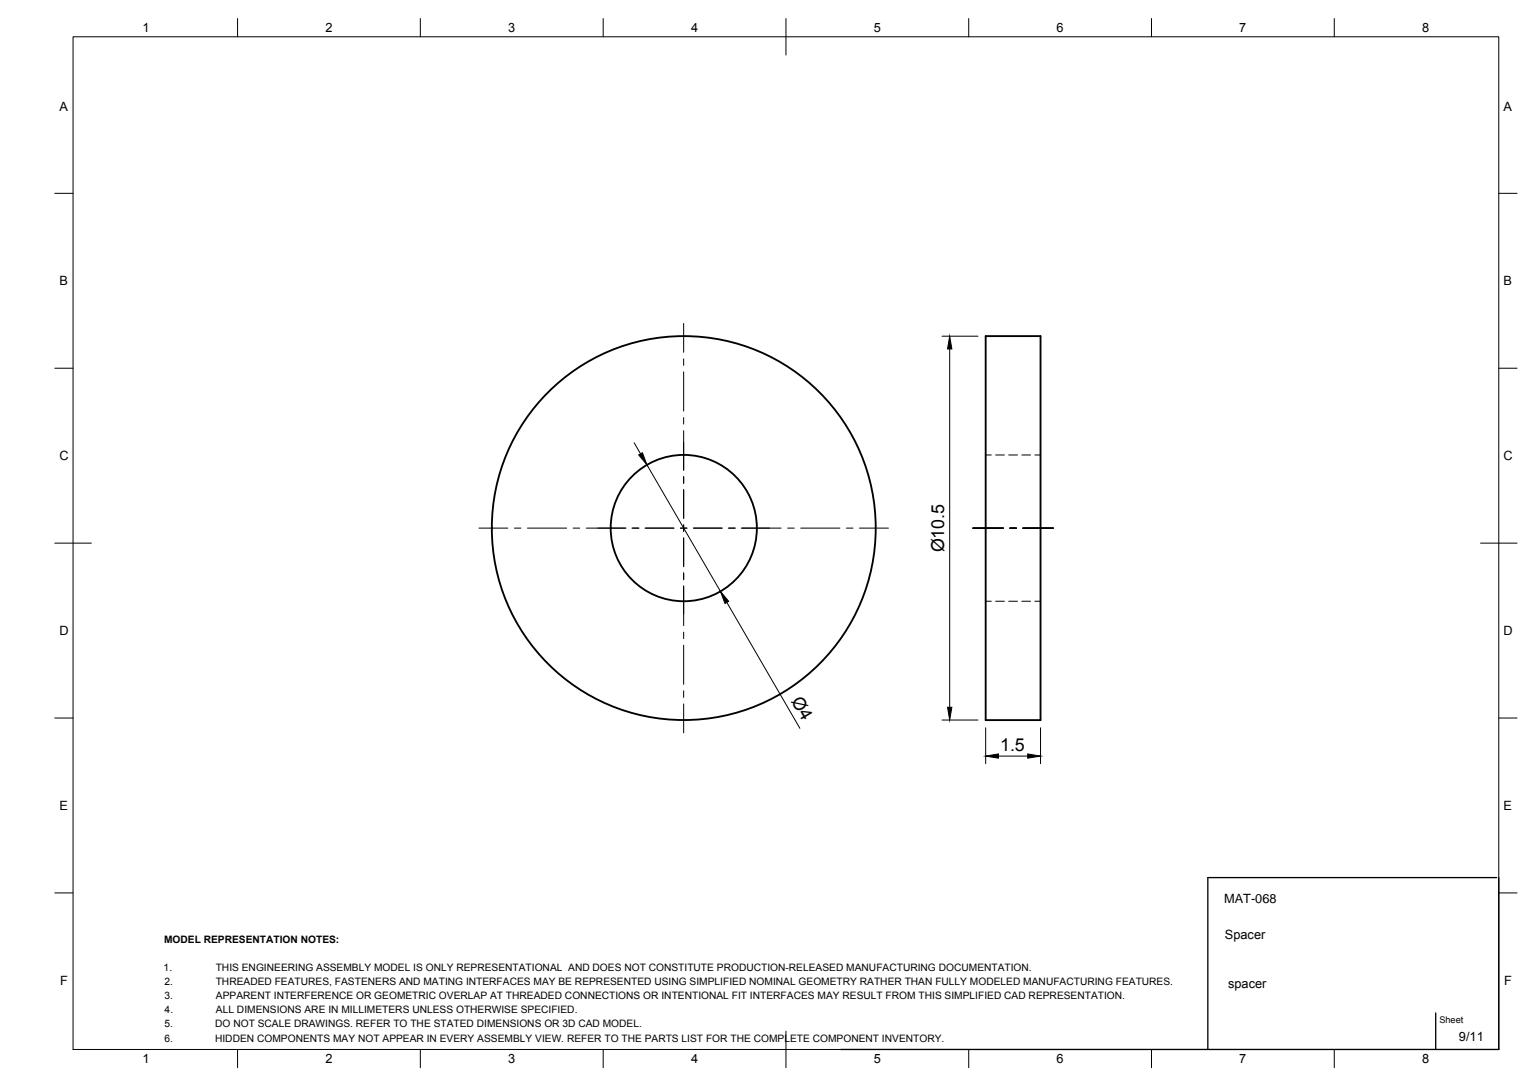
ISO-10303-21;
HEADER;
/* Generated by software containing ST-Developer
 * from STEP Tools, Inc. (www.steptools.com) 
 */

FILE_DESCRIPTION(
/* description */ ('CAx-IF Rec.Pracs.---Representation and Presentation of Product Manufa
cturing Information (PMI)---4.0---2014-10-13'),
/* implementation_level */ '2;1');

FILE_NAME(
/* name */ 'Spacer.step',
/* time_stamp */ '2026-10-24T16:53:48-07:00',
/* author */ (''),
/* organization */ (''),
/* preprocessor_version */ 'ST-DEVELOPER v20.2',
/* originating_system */ 'Autodesk Translation Framework v15.17.0.0',
/* authorisation */ '');

FILE_SCHEMA (('AP242_MANAGED_MODEL_BASED_3D_ENGINEERING_MIM_LF { 1 0 10303 442 2 1 4 }'));
ENDSEC;

DATA;
#10=MECHANICAL_DESIGN_GEOMETRIC_PRESENTATION_REPRESENTATION('',(#3496),#107910);
#3476=SHAPE_REPRESENTATION_RELATIONSHIP('SRR','None',#107954,#3486);
#3486=ADVANCED_BREP_SHAPE_REPRESENTATION('',(#3506),#107907);
#3496=STYLED_ITEM('',(#108011),#3506);
#3506=MANIFOLD_SOLID_BREP('Body1',#45544);
#3517=FACE_BOUND('',#9340,.T.);
#3518=FACE_BOUND('',#9342,.T.);
#3572=PLANE('',#49897);
#3573=PLANE('',#49898);
#6405=FACE_OUTER_BOUND('',#9337,.T.);
#6406=FACE_OUTER_BOUND('',#9338,.T.);
#6407=FACE_OUTER_BOUND('',#9339,.T.);
#6408=FACE_OUTER_BOUND('',#9341,.T.);
#9337=EDGE_LOOP('',(#40400,#40401,#40402,#40403));
#9338=EDGE_LOOP('',(#40404,#40405,#40406,#40407));
#9339=EDGE_LOOP('',(#40408));
#9340=EDGE_LOOP('',(#40409));
#9341=EDGE_LOOP('',(#40410));
#9342=EDGE_LOOP('',(#40411));
#11042=LINE('',#106251,#13026);
#11043=LINE('',#106257,#13027);
#13026=VECTOR('',#60249,0.002);
#13027=VECTOR('',#60256,0.00525);
#16983=CIRCLE('',#49892,0.00200000000001);
#16984=CIRCLE('',#49893,0.00200000000001);
#16985=CIRCLE('',#49895,0.00525000000001);
#16986=CIRCLE('',#49896,0.00525000000001);
#20687=VERTEX_POINT('',#106248);
#20688=VERTEX_POINT('',#106250);
#20689=VERTEX_POINT('',#106254);
#20690=VERTEX_POINT('',#106256);
#27342=EDGE_CURVE('',#20687,#20687,#16983,.T.);
#27343=EDGE_CURVE('',#20687,#20688,#11042,.T.);
#27344=EDGE_CURVE('',#20688,#20688,#16984,.T.);
#27345=EDGE_CURVE('',#20689,#20689,#16985,.T.);
#27346=EDGE_CURVE('',#20689,#20690,#11043,.T.);
#27347=EDGE_CURVE('',#20690,#20690,#16986,.T.);
#40400=ORIENTED_EDGE('',*,*,#27342,.F.);
#40401=ORIENTED_EDGE('',*,*,#27343,.T.);
#40402=ORIENTED_EDGE('',*,*,#27344,.T.);
#40403=ORIENTED_EDGE('',*,*,#27343,.F.);
#40404=ORIENTED_EDGE('',*,*,#27345,.T.);
#40405=ORIENTED_EDGE('',*,*,#27346,.T.);
#40406=ORIENTED_EDGE('',*,*,#27347,.F.);
#40407=ORIENTED_EDGE('',*,*,#27346,.F.);
#40408=ORIENTED_EDGE('',*,*,#27347,.T.);
#40409=ORIENTED_EDGE('',*,*,#27344,.F.);
#40410=ORIENTED_EDGE('',*,*,#27345,.F.);
#40411=ORIENTED_EDGE('',*,*,#27342,.T.);
#42523=CYLINDRICAL_SURFACE('',#49891,0.002);
#42524=CYLINDRICAL_SURFACE('',#49894,0.00525);
#45260=ADVANCED_FACE('',(#6405),#42523,.F.);
#45261=ADVANCED_FACE('',(#6406),#42524,.T.);
#45262=ADVANCED_FACE('',(#6407,#3517),#3572,.T.);
#45263=ADVANCED_FACE('',(#6408,#3518),#3573,.F.);
#45544=CLOSED_SHELL('',(#45260,#45261,#45262,#45263));
#49890=AXIS2_PLACEMENT_3D('',#106246,#60243,#60244);
#49891=AXIS2_PLACEMENT_3D('',#106247,#60245,#60246);
#49892=AXIS2_PLACEMENT_3D('',#106249,#60247,#60248);
#49893=AXIS2_PLACEMENT_3D('',#106252,#60250,#60251);
#49894=AXIS2_PLACEMENT_3D('',#106253,#60252,#60253);
#49895=AXIS2_PLACEMENT_3D('',#106255,#60254,#60255);
#49896=AXIS2_PLACEMENT_3D('',#106258,#60257,#60258);
#49897=AXIS2_PLACEMENT_3D('',#106259,#60259,#60260);
#49898=AXIS2_PLACEMENT_3D('',#106260,#60261,#60262);
#60243=DIRECTION('axis',(0.,0.,1.));
#60244=DIRECTION('refdir',(1.,0.,0.));
#60245=DIRECTION('center_axis',(1.,0.,0.));
#60246=DIRECTION('ref_axis',(0.,0.,-1.));
#60247=DIRECTION('center_axis',(1.,0.,0.));
#60248=DIRECTION('ref_axis',(0.,0.,-1.));
#60249=DIRECTION('',(1.,0.,0.));
#60250=DIRECTION('center_axis',(1.,0.,0.));
#60251=DIRECTION('ref_axis',(0.,0.,-1.));
#60252=DIRECTION('center_axis',(-1.,0.,0.));
#60253=DIRECTION('ref_axis',(0.,0.,1.));
#60254=DIRECTION('center_axis',(1.,0.,0.));
#60255=DIRECTION('ref_axis',(0.,0.,-1.));
#60256=DIRECTION('',(1.,0.,0.));
#60257=DIRECTION('center_axis',(1.,0.,0.));
#60258=DIRECTION('ref_axis',(0.,0.,-1.));
#60259=DIRECTION('center_axis',(1.,0.,0.));
#60260=DIRECTION('ref_axis',(0.,1.,0.));
#60261=DIRECTION('center_axis',(1.,0.,0.));
#60262=DIRECTION('ref_axis',(0.,1.,0.));
#106246=CARTESIAN_POINT('',(0.,0.,0.));
#106247=CARTESIAN_POINT('Origin',(-0.0411262178068916,-0.00152418147196182,
0.079));
#106248=CARTESIAN_POINT('',(0.0121237821931184,-0.00152418147196182,0.081));
#106249=CARTESIAN_POINT('Origin',(0.0121237821931184,-0.00152418147197183,
0.07900000000001));
#106250=CARTESIAN_POINT('',(0.0136237821931184,-0.00152418147196182,0.081));
#106251=CARTESIAN_POINT('',(-0.0411262178068916,-0.00152418147196182,0.081));
#106252=CARTESIAN_POINT('Origin',(0.0136237821931184,-0.00152418147197183,
0.07900000000001));
#106253=CARTESIAN_POINT('Origin',(0.0136237821931084,-0.00152418147196182,
0.079));
#106254=CARTESIAN_POINT('',(0.0121237821931184,-0.00152418147197183,0.07375));
#106255=CARTESIAN_POINT('Origin',(0.0121237821931184,-0.00152418147197183,
0.07900000000001));
#106256=CARTESIAN_POINT('',(0.0136237821931184,-0.00152418147197183,0.07375));
#106257=CARTESIAN_POINT('',(0.0136237821931084,-0.00152418147196182,0.07375));
#106258=CARTESIAN_POINT('Origin',(0.0136237821931184,-0.00152418147197183,
0.07900000000001));
#106259=CARTESIAN_POINT('Origin',(0.0136237821931084,-0.00152418147196182,
0.079));
#106260=CARTESIAN_POINT('Origin',(0.0121237821931084,-0.00152418147196182,
0.079));
#107895=UNCERTAINTY_MEASURE_WITH_UNIT(LENGTH_MEASURE(1.E-5),#107911,
'DISTANCE_ACCURACY_VALUE',
'Maximum model space distance between geometric entities at asserted c
onnectivities');
#107898=UNCERTAINTY_MEASURE_WITH_UNIT(LENGTH_MEASURE(1.E-5),#107911,
'DISTANCE_ACCURACY_VALUE',
'Maximum model space distance between geometric entities at asserted c
onnectivities');
#107907=(
GEOMETRIC_REPRESENTATION_CONTEXT(3)
GLOBAL_UNCERTAINTY_ASSIGNED_CONTEXT((#107895))
GLOBAL_UNIT_ASSIGNED_CONTEXT((#107911,#107912,#107913))
REPRESENTATION_CONTEXT('','3D')
);
#107910=(
GEOMETRIC_REPRESENTATION_CONTEXT(3)
GLOBAL_UNCERTAINTY_ASSIGNED_CONTEXT((#107898))
GLOBAL_UNIT_ASSIGNED_CONTEXT((#107911,#107912,#107913))
REPRESENTATION_CONTEXT('','3D')
);
#107911=(
LENGTH_UNIT()
NAMED_UNIT(*)
SI_UNIT($,.METRE.)
);
#107912=(
NAMED_UNIT(*)
PLANE_ANGLE_UNIT()
SI_UNIT($,.RADIAN.)
);
#107913=(
NAMED_UNIT(*)
SI_UNIT($,.STERADIAN.)
SOLID_ANGLE_UNIT()
);
#107922=SHAPE_DEFINITION_REPRESENTATION(#107933,#107954);
#107933=PRODUCT_DEFINITION_SHAPE('',$,#107966);
#107954=SHAPE_REPRESENTATION('',(#49890),#107907);
#107957=PRODUCT_DEFINITION_CONTEXT('part definition',#107992,'design');
#107966=PRODUCT_DEFINITION('Spacer','Spacer',#107977,#107957);
#107977=PRODUCT_DEFINITION_FORMATION('',$,#108002);
#107992=APPLICATION_CONTEXT('Managed model based 3d engineering');
#107993=PRODUCT_CONTEXT('part definition',#107992,'mechanical');
#108002=PRODUCT('Spacer','Spacer',
'LEGAL AND USAGE DISCLAIMER: this Data/Model is provided \X2\201C\X0\A
S IS\X2\201D\X0\ for informational and representational only. It is a 
geometric approximation and is NOT engineered, certified, or guarantee
d for dimensional accuracy, exact tolerances, or production-level prec
ision. Vendor disclaims all implied warranties including fitness for a
 particular purpose. DO NOT USE FOR DIRECT PHYSICAL MANUFACTURING, AUT
OMATED PRODUCTION, OR SAFETY-CRITICAL SYSTEMS without independent engi
neering verification and resolution of any design discrepancies.',(#107993));
#108011=PRESENTATION_STYLE_ASSIGNMENT((#108018));
#108018=SURFACE_STYLE_USAGE(.BOTH.,#108025);
#108025=SURFACE_SIDE_STYLE('',(#108032));
#108032=SURFACE_STYLE_FILL_AREA(#108039);
#108039=FILL_AREA_STYLE('Opaque(137,137,137)',(#108046));
#108046=FILL_AREA_STYLE_COLOUR('Opaque(137,137,137)',#108053);
#108053=COLOUR_RGB('Opaque(137,137,137)',0.537254901960784,0.537254901960784,
0.537254901960784);
ENDSEC;
END-ISO-10303-21;
